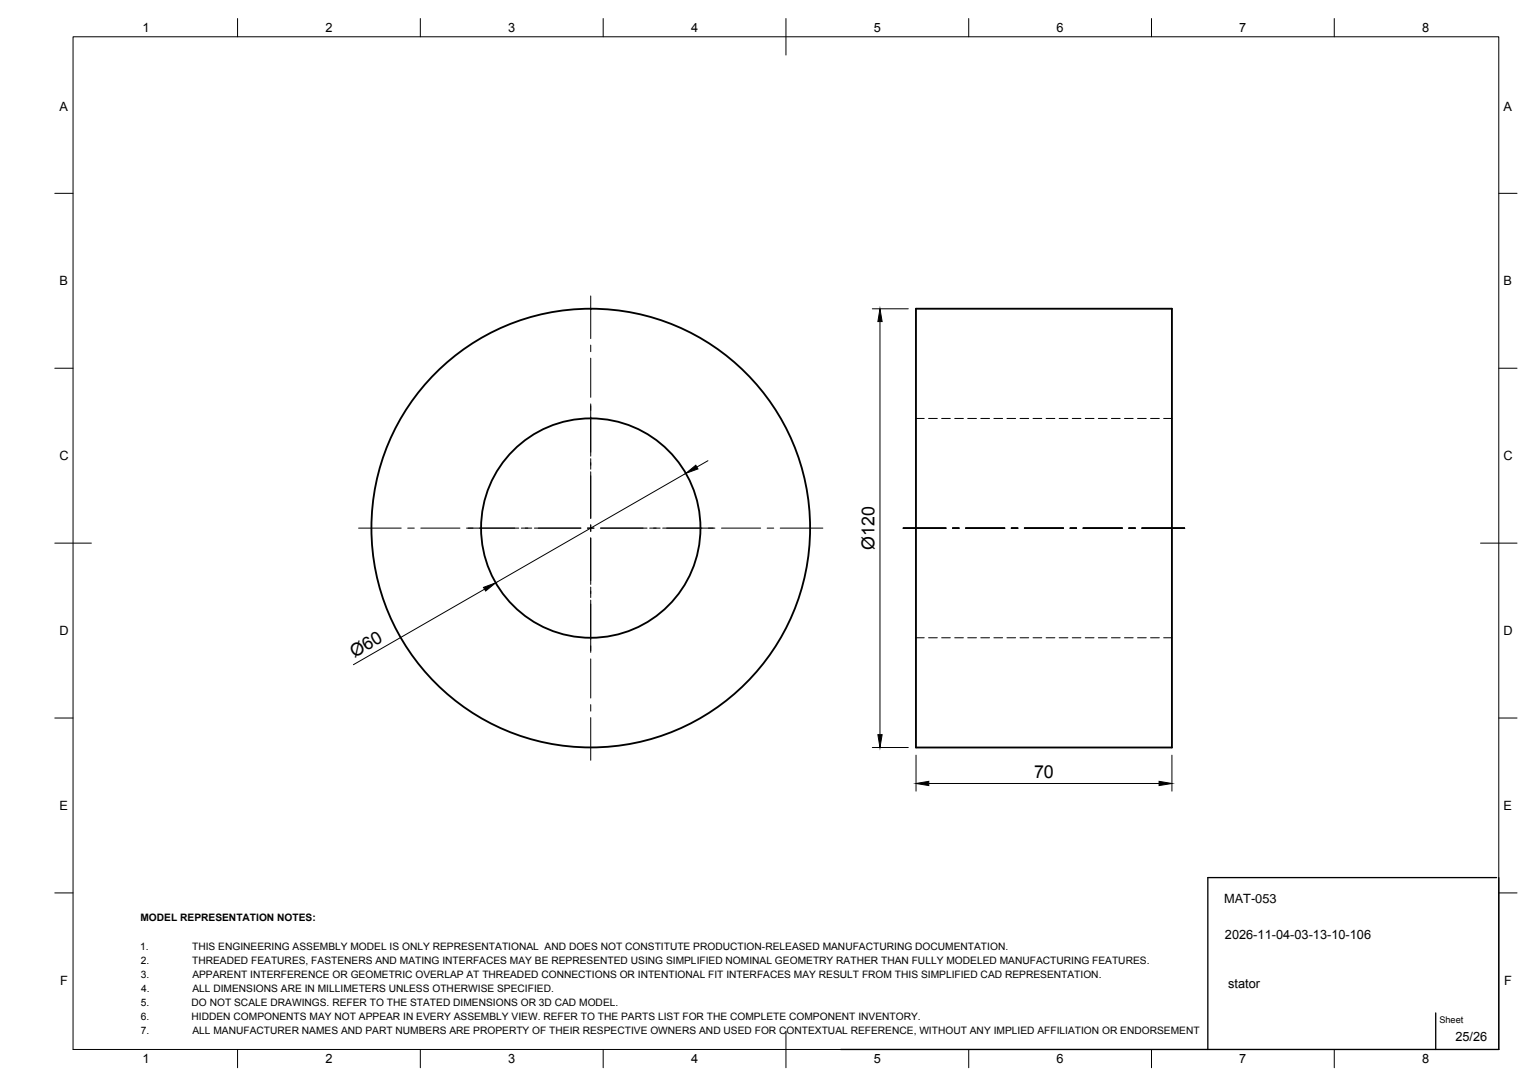
ISO-10303-21;
HEADER;
FILE_DESCRIPTION (('STEP AP214'),
    '1' );
FILE_NAME ('stator.step',
    '2026-10-10T03:43:58',
    ( '' ),
    ( '' ),
    'SwSTEP 2.0',
    'SolidWorks 2026',
    '' );
FILE_SCHEMA (( 'AUTOMOTIVE_DESIGN' ));
ENDSEC;

DATA;
#128=EDGE_CURVE ( 'NONE', #3129, #8050, #2808, .T. ) ;
#514=DIRECTION ( 'NONE',  ( 0.000000000000000000, 0.000000000000000000, -1.000000000000000000 ) ) ;
#771=EDGE_LOOP ( 'NONE', ( #32204, #20972 ) ) ;
#1378=ORIENTED_EDGE ( 'NONE', *, *, #27790, .F. ) ;
#2079=CARTESIAN_POINT ( 'NONE',  ( 0.000000000000000000, 70.00000000000000000, 0.000000000000000000 ) ) ;
#2691=DIRECTION ( 'NONE',  ( 0.000000000000000000, -0.000000000000000000, 1.000000000000000000 ) ) ;
#2808=LINE ( 'NONE', #13704, #47364 ) ;
#2968=ORIENTED_EDGE ( 'NONE', *, *, #54046, .T. ) ;
#3097=DIRECTION ( 'NONE',  ( 1.000000000000000000, 0.000000000000000000, 0.000000000000000000 ) ) ;
#3129=VERTEX_POINT ( 'NONE', #8923 ) ;
#3877=CARTESIAN_POINT ( 'NONE',  ( 0.000000000000000000, 70.00000000000000000, 0.000000000000000000 ) ) ;
#3906=VERTEX_POINT ( 'NONE', #13515 ) ;
#5010=PRODUCT_DEFINITION_CONTEXT ( 'detailed design', #48477, 'design' ) ;
#5620=SURFACE_STYLE_FILL_AREA ( #37284 ) ;
#6322=( NAMED_UNIT ( * ) SI_UNIT ( $, .STERADIAN. ) SOLID_ANGLE_UNIT ( ) );
#6922=DIRECTION ( 'NONE',  ( 0.000000000000000000, 0.000000000000000000, 1.000000000000000000 ) ) ;
#7111=DIRECTION ( 'NONE',  ( 0.000000000000000000, 1.000000000000000000, 0.000000000000000000 ) ) ;
#7237=ORIENTED_EDGE ( 'NONE', *, *, #40186, .F. ) ;
#7402=EDGE_CURVE ( 'NONE', #11928, #12092, #39946, .T. ) ;
#7531=CARTESIAN_POINT ( 'NONE',  ( 0.000000000000000000, 0.000000000000000000, -60.00000000000000000 ) ) ;
#8050=VERTEX_POINT ( 'NONE', #9236 ) ;
#8164=AXIS2_PLACEMENT_3D ( 'NONE', #38494, #11061, #514 ) ;
#8303=ORIENTED_EDGE ( 'NONE', *, *, #10070, .T. ) ;
#8319=DIRECTION ( 'NONE',  ( 1.000000000000000000, 0.000000000000000000, 0.000000000000000000 ) ) ;
#8479=CARTESIAN_POINT ( 'NONE',  ( 3.673940397442059178E-15, 70.00000000000000000, 30.00000000000000000 ) ) ;
#8923=CARTESIAN_POINT ( 'NONE',  ( 7.347880794884118356E-15, 70.00000000000000000, 60.00000000000000000 ) ) ;
#9236=CARTESIAN_POINT ( 'NONE',  ( 7.347880794884118356E-15, 0.000000000000000000, 60.00000000000000000 ) ) ;
#10070=EDGE_CURVE ( 'NONE', #11364, #8050, #65973, .T. ) ;
#10554=FILL_AREA_STYLE_COLOUR ( '', #23478 ) ;
#10805=PRODUCT_DEFINITION_FORMATION_WITH_SPECIFIED_SOURCE ( 'ANY', '', #45703, .NOT_KNOWN. ) ;
#11061=DIRECTION ( 'NONE',  ( -0.000000000000000000, -1.000000000000000000, -0.000000000000000000 ) ) ;
#11364=VERTEX_POINT ( 'NONE', #7531 ) ;
#11398=CYLINDRICAL_SURFACE ( 'NONE', #8164, 60.00000000000000000 ) ;
#11411=CLOSED_SHELL ( 'NONE', ( #11814, #48594, #51527, #41201, #53636, #22060 ) ) ;
#11814=ADVANCED_FACE ( 'NONE', ( #47465 ), #57354, .F. ) ;
#11928=VERTEX_POINT ( 'NONE', #8479 ) ;
#12092=VERTEX_POINT ( 'NONE', #18597 ) ;
#12606=ORIENTED_EDGE ( 'NONE', *, *, #34401, .T. ) ;
#13254=FACE_OUTER_BOUND ( 'NONE', #69197, .T. ) ;
#13515=CARTESIAN_POINT ( 'NONE',  ( 0.000000000000000000, 70.00000000000000000, -60.00000000000000000 ) ) ;
#13591=DIRECTION ( 'NONE',  ( 0.000000000000000000, 1.000000000000000000, 0.000000000000000000 ) ) ;
#13704=CARTESIAN_POINT ( 'NONE',  ( 7.347880794884118356E-15, 70.00000000000000000, 60.00000000000000000 ) ) ;
#13722=DIRECTION ( 'NONE',  ( 0.000000000000000000, 1.000000000000000000, 0.000000000000000000 ) ) ;
#14303=ORIENTED_EDGE ( 'NONE', *, *, #34401, .F. ) ;
#14387=CARTESIAN_POINT ( 'NONE',  ( 0.000000000000000000, 70.00000000000000000, -30.00000000000000000 ) ) ;
#15284=DIRECTION ( 'NONE',  ( 0.000000000000000000, 1.000000000000000000, 0.000000000000000000 ) ) ;
#15336=EDGE_CURVE ( 'NONE', #12092, #11928, #55552, .T. ) ;
#16532=AXIS2_PLACEMENT_3D ( 'NONE', #62277, #31318, #62972 ) ;
#16657=AXIS2_PLACEMENT_3D ( 'NONE', #26661, #63948, #26322 ) ;
#17905=AXIS2_PLACEMENT_3D ( 'NONE', #34759, #57593, #3097 ) ;
#17988=ORIENTED_EDGE ( 'NONE', *, *, #58843, .T. ) ;
#18093=( LENGTH_UNIT ( ) NAMED_UNIT ( * ) SI_UNIT ( .MILLI., .METRE. ) );
#18597=CARTESIAN_POINT ( 'NONE',  ( 0.000000000000000000, 70.00000000000000000, -30.00000000000000000 ) ) ;
#19703=( GEOMETRIC_REPRESENTATION_CONTEXT ( 3 ) GLOBAL_UNCERTAINTY_ASSIGNED_CONTEXT ( ( #55717 ) ) GLOBAL_UNIT_ASSIGNED_CONTEXT ( ( #18093, #66306, #23020 ) ) REPRESENTATION_CONTEXT ( 'NONE', 'WORKASPACE' ) );
#19882=EDGE_LOOP ( 'NONE', ( #42252, #31669, #65286, #8303 ) ) ;
#19919=EDGE_LOOP ( 'NONE', ( #40783, #67233 ) ) ;
#20062=ORIENTED_EDGE ( 'NONE', *, *, #128, .T. ) ;
#20100=MECHANICAL_DESIGN_GEOMETRIC_PRESENTATION_REPRESENTATION('',(#40332),#38058);
#20972=ORIENTED_EDGE ( 'NONE', *, *, #7402, .F. ) ;
#21799=PRESENTATION_STYLE_ASSIGNMENT (( #53454 ) ) ;
#22060=ADVANCED_FACE ( 'NONE', ( #55522 ), #50256, .F. ) ;
#23020=( NAMED_UNIT ( * ) SI_UNIT ( $, .STERADIAN. ) SOLID_ANGLE_UNIT ( ) );
#23025=AXIS2_PLACEMENT_3D ( 'NONE', #33668, #55448, #6922 ) ;
#23478=COLOUR_RGB ( '',0.7921568627450980005, 0.8196078431372548767, 0.9333333333333333481 ) ;
#23530=DIRECTION ( 'NONE',  ( -0.000000000000000000, -1.000000000000000000, -0.000000000000000000 ) ) ;
#23730=DIRECTION ( 'NONE',  ( -0.000000000000000000, -1.000000000000000000, -0.000000000000000000 ) ) ;
#25005=LINE ( 'NONE', #35552, #56810 ) ;
#25560=VERTEX_POINT ( 'NONE', #41893 ) ;
#25651=ORIENTED_EDGE ( 'NONE', *, *, #27790, .T. ) ;
#26071=CARTESIAN_POINT ( 'NONE',  ( 3.673940397442059178E-15, 0.000000000000000000, 30.00000000000000000 ) ) ;
#26322=DIRECTION ( 'NONE',  ( 0.000000000000000000, 0.000000000000000000, -1.000000000000000000 ) ) ;
#26661=CARTESIAN_POINT ( 'NONE',  ( 0.000000000000000000, 70.00000000000000000, 0.000000000000000000 ) ) ;
#26809=ORIENTED_EDGE ( 'NONE', *, *, #49285, .F. ) ;
#27752=AXIS2_PLACEMENT_3D ( 'NONE', #29958, #7111, #51420 ) ;
#27790=EDGE_CURVE ( 'NONE', #11928, #65701, #25005, .T. ) ;
#28733=PLANE ( 'NONE',  #66663 ) ;
#29336=SHAPE_REPRESENTATION_RELATIONSHIP ( 'NONE' , 'NONE' ,  #38847, #62542 ) ;
#29349=LINE ( 'NONE', #61013, #40185 ) ;
#29675=UNCERTAINTY_MEASURE_WITH_UNIT (LENGTH_MEASURE( 1.000000000000000082E-05 ), #49218, 'distance_accuracy_value', 'NONE');
#29958=CARTESIAN_POINT ( 'NONE',  ( 0.000000000000000000, 0.000000000000000000, 0.000000000000000000 ) ) ;
#30601=CARTESIAN_POINT ( 'NONE',  ( 0.000000000000000000, 70.00000000000000000, 0.000000000000000000 ) ) ;
#31318=DIRECTION ( 'NONE',  ( -0.000000000000000000, -1.000000000000000000, -0.000000000000000000 ) ) ;
#31350=EDGE_CURVE ( 'NONE', #3906, #11364, #29349, .T. ) ;
#31410=CIRCLE ( 'NONE', #17905, 60.00000000000000000 ) ;
#31669=ORIENTED_EDGE ( 'NONE', *, *, #52351, .F. ) ;
#31674=( NAMED_UNIT ( * ) PLANE_ANGLE_UNIT ( ) SI_UNIT ( $, .RADIAN. ) );
#32204=ORIENTED_EDGE ( 'NONE', *, *, #15336, .F. ) ;
#32372=SURFACE_SIDE_STYLE ('',( #5620 ) ) ;
#32497=CARTESIAN_POINT ( 'NONE',  ( 0.000000000000000000, 0.000000000000000000, 0.000000000000000000 ) ) ;
#32994=CIRCLE ( 'NONE', #47593, 30.00000000000000000 ) ;
#33668=CARTESIAN_POINT ( 'NONE',  ( 0.000000000000000000, 70.00000000000000000, 0.000000000000000000 ) ) ;
#34275=CIRCLE ( 'NONE', #66872, 60.00000000000000000 ) ;
#34401=EDGE_CURVE ( 'NONE', #3129, #3906, #31410, .T. ) ;
#34759=CARTESIAN_POINT ( 'NONE',  ( 0.000000000000000000, 70.00000000000000000, 0.000000000000000000 ) ) ;
#35552=CARTESIAN_POINT ( 'NONE',  ( 3.673940397442059178E-15, 70.00000000000000000, 30.00000000000000000 ) ) ;
#36639=ORIENTED_EDGE ( 'NONE', *, *, #31350, .F. ) ;
#36743=CARTESIAN_POINT ( 'NONE',  ( 0.000000000000000000, 0.000000000000000000, 0.000000000000000000 ) ) ;
#36757=CIRCLE ( 'NONE', #27752, 30.00000000000000000 ) ;
#36786=AXIS2_PLACEMENT_3D ( 'NONE', #36743, #15284, #62438 ) ;
#36923=DIRECTION ( 'NONE',  ( 1.000000000000000000, 0.000000000000000000, 0.000000000000000000 ) ) ;
#37284=FILL_AREA_STYLE ('',( #10554 ) ) ;
#37524=CARTESIAN_POINT ( 'NONE',  ( 0.000000000000000000, 0.000000000000000000, 0.000000000000000000 ) ) ;
#37638=ORIENTED_EDGE ( 'NONE', *, *, #15336, .T. ) ;
#38058=( GEOMETRIC_REPRESENTATION_CONTEXT ( 3 ) GLOBAL_UNCERTAINTY_ASSIGNED_CONTEXT ( ( #29675 ) ) GLOBAL_UNIT_ASSIGNED_CONTEXT ( ( #49218, #31674, #6322 ) ) REPRESENTATION_CONTEXT ( 'NONE', 'WORKASPACE' ) );
#38494=CARTESIAN_POINT ( 'NONE',  ( 0.000000000000000000, 70.00000000000000000, 0.000000000000000000 ) ) ;
#38847=SHAPE_REPRESENTATION ( 'stator', ( #66832 ), #19703 ) ;
#38996=ORIENTED_EDGE ( 'NONE', *, *, #7402, .T. ) ;
#39079=FACE_OUTER_BOUND ( 'NONE', #44402, .T. ) ;
#39696=VECTOR ( 'NONE', #50973, 1000.000000000000000 ) ;
#39764=PLANE ( 'NONE',  #42835 ) ;
#39946=CIRCLE ( 'NONE', #59011, 30.00000000000000000 ) ;
#40136=DIRECTION ( 'NONE',  ( -0.000000000000000000, -1.000000000000000000, -0.000000000000000000 ) ) ;
#40185=VECTOR ( 'NONE', #23730, 1000.000000000000000 ) ;
#40186=EDGE_CURVE ( 'NONE', #65701, #25560, #32994, .T. ) ;
#40332=STYLED_ITEM ( 'NONE', ( #21799 ), #64301 ) ;
#40783=ORIENTED_EDGE ( 'NONE', *, *, #49285, .T. ) ;
#41023=SHAPE_DEFINITION_REPRESENTATION ( #55202, #38847 ) ;
#41201=ADVANCED_FACE ( 'NONE', ( #13254, #61086 ), #28733, .F. ) ;
#41893=CARTESIAN_POINT ( 'NONE',  ( 0.000000000000000000, 0.000000000000000000, -30.00000000000000000 ) ) ;
#42252=ORIENTED_EDGE ( 'NONE', *, *, #128, .F. ) ;
#42699=DIRECTION ( 'NONE',  ( 0.000000000000000000, 1.000000000000000000, 0.000000000000000000 ) ) ;
#42835=AXIS2_PLACEMENT_3D ( 'NONE', #65818, #13722, #50660 ) ;
#43080=PRODUCT_DEFINITION ( 'UNKNOWN', '', #10805, #5010 ) ;
#43081=AXIS2_PLACEMENT_3D ( 'NONE', #2079, #23530, #45318 ) ;
#43167=CYLINDRICAL_SURFACE ( 'NONE', #16657, 60.00000000000000000 ) ;
#43193=ORIENTED_EDGE ( 'NONE', *, *, #54046, .F. ) ;
#44402=EDGE_LOOP ( 'NONE', ( #67755, #12606 ) ) ;
#44558=DIRECTION ( 'NONE',  ( 0.000000000000000000, 0.000000000000000000, 1.000000000000000000 ) ) ;
#44655=ORIENTED_EDGE ( 'NONE', *, *, #10070, .F. ) ;
#45318=DIRECTION ( 'NONE',  ( 0.000000000000000000, 0.000000000000000000, -1.000000000000000000 ) ) ;
#45703=PRODUCT ( 'stator', 'stator', '', ( #47664 ) ) ;
#46417=EDGE_LOOP ( 'NONE', ( #37638, #25651, #26809, #43193 ) ) ;
#47364=VECTOR ( 'NONE', #67195, 1000.000000000000000 ) ;
#47465=FACE_OUTER_BOUND ( 'NONE', #46417, .T. ) ;
#47593=AXIS2_PLACEMENT_3D ( 'NONE', #37524, #65310, #54384 ) ;
#47664=PRODUCT_CONTEXT ( 'NONE', #66008, 'mechanical' ) ;
#47809=DIRECTION ( 'NONE',  ( 0.000000000000000000, 1.000000000000000000, 0.000000000000000000 ) ) ;
#48477=APPLICATION_CONTEXT ( 'automotive_design' ) ;
#48496=CIRCLE ( 'NONE', #57529, 60.00000000000000000 ) ;
#48594=ADVANCED_FACE ( 'NONE', ( #53723 ), #43167, .T. ) ;
#49218=( LENGTH_UNIT ( ) NAMED_UNIT ( * ) SI_UNIT ( .MILLI., .METRE. ) );
#49285=EDGE_CURVE ( 'NONE', #25560, #65701, #36757, .T. ) ;
#50256=CYLINDRICAL_SURFACE ( 'NONE', #43081, 30.00000000000000000 ) ;
#50530=CARTESIAN_POINT ( 'NONE',  ( 0.000000000000000000, 0.000000000000000000, 0.000000000000000000 ) ) ;
#50660=DIRECTION ( 'NONE',  ( 0.000000000000000000, -0.000000000000000000, 1.000000000000000000 ) ) ;
#50973=DIRECTION ( 'NONE',  ( -0.000000000000000000, -1.000000000000000000, -0.000000000000000000 ) ) ;
#51420=DIRECTION ( 'NONE',  ( 0.000000000000000000, 0.000000000000000000, 1.000000000000000000 ) ) ;
#51527=ADVANCED_FACE ( 'NONE', ( #39079, #55588 ), #39764, .T. ) ;
#52351=EDGE_CURVE ( 'NONE', #3906, #3129, #48496, .T. ) ;
#53454=SURFACE_STYLE_USAGE ( .BOTH. , #32372 ) ;
#53588=DIRECTION ( 'NONE',  ( 1.000000000000000000, 0.000000000000000000, 0.000000000000000000 ) ) ;
#53636=ADVANCED_FACE ( 'NONE', ( #65953 ), #11398, .T. ) ;
#53723=FACE_OUTER_BOUND ( 'NONE', #67488, .T. ) ;
#54046=EDGE_CURVE ( 'NONE', #12092, #25560, #56950, .T. ) ;
#54384=DIRECTION ( 'NONE',  ( 0.000000000000000000, 0.000000000000000000, 1.000000000000000000 ) ) ;
#55202=PRODUCT_DEFINITION_SHAPE ( 'NONE', 'NONE',  #43080 ) ;
#55448=DIRECTION ( 'NONE',  ( 0.000000000000000000, 1.000000000000000000, 0.000000000000000000 ) ) ;
#55522=FACE_OUTER_BOUND ( 'NONE', #66699, .T. ) ;
#55552=CIRCLE ( 'NONE', #23025, 30.00000000000000000 ) ;
#55588=FACE_BOUND ( 'NONE', #771, .T. ) ;
#55717=UNCERTAINTY_MEASURE_WITH_UNIT (LENGTH_MEASURE( 1.000000000000000082E-05 ), #18093, 'distance_accuracy_value', 'NONE');
#56635=DIRECTION ( 'NONE',  ( 0.000000000000000000, 1.000000000000000000, 0.000000000000000000 ) ) ;
#56810=VECTOR ( 'NONE', #40136, 1000.000000000000000 ) ;
#56950=LINE ( 'NONE', #14387, #39696 ) ;
#57354=CYLINDRICAL_SURFACE ( 'NONE', #16532, 30.00000000000000000 ) ;
#57529=AXIS2_PLACEMENT_3D ( 'NONE', #3877, #47809, #36923 ) ;
#57593=DIRECTION ( 'NONE',  ( 0.000000000000000000, 1.000000000000000000, 0.000000000000000000 ) ) ;
#58843=EDGE_CURVE ( 'NONE', #8050, #11364, #34275, .T. ) ;
#59011=AXIS2_PLACEMENT_3D ( 'NONE', #30601, #56635, #66866 ) ;
#59446=ORIENTED_EDGE ( 'NONE', *, *, #58843, .F. ) ;
#61013=CARTESIAN_POINT ( 'NONE',  ( 0.000000000000000000, 70.00000000000000000, -60.00000000000000000 ) ) ;
#61086=FACE_BOUND ( 'NONE', #19919, .T. ) ;
#61765=CARTESIAN_POINT ( 'NONE',  ( 0.000000000000000000, 0.000000000000000000, 0.000000000000000000 ) ) ;
#62277=CARTESIAN_POINT ( 'NONE',  ( 0.000000000000000000, 70.00000000000000000, 0.000000000000000000 ) ) ;
#62438=DIRECTION ( 'NONE',  ( 1.000000000000000000, 0.000000000000000000, 0.000000000000000000 ) ) ;
#62542=ADVANCED_BREP_SHAPE_REPRESENTATION ( '', ( #64301, #66832 ), #19703 ) ;
#62972=DIRECTION ( 'NONE',  ( 0.000000000000000000, 0.000000000000000000, -1.000000000000000000 ) ) ;
#63948=DIRECTION ( 'NONE',  ( -0.000000000000000000, -1.000000000000000000, -0.000000000000000000 ) ) ;
#64301=MANIFOLD_SOLID_BREP ( 'Extrude-Thin1', #11411 ) ;
#65286=ORIENTED_EDGE ( 'NONE', *, *, #31350, .T. ) ;
#65310=DIRECTION ( 'NONE',  ( 0.000000000000000000, 1.000000000000000000, 0.000000000000000000 ) ) ;
#65701=VERTEX_POINT ( 'NONE', #26071 ) ;
#65818=CARTESIAN_POINT ( 'NONE',  ( 0.000000000000000000, 70.00000000000000000, 0.000000000000000000 ) ) ;
#65953=FACE_OUTER_BOUND ( 'NONE', #19882, .T. ) ;
#65973=CIRCLE ( 'NONE', #36786, 60.00000000000000000 ) ;
#66008=APPLICATION_CONTEXT ( 'automotive_design' ) ;
#66306=( NAMED_UNIT ( * ) PLANE_ANGLE_UNIT ( ) SI_UNIT ( $, .RADIAN. ) );
#66663=AXIS2_PLACEMENT_3D ( 'NONE', #61765, #13591, #2691 ) ;
#66699=EDGE_LOOP ( 'NONE', ( #1378, #38996, #2968, #7237 ) ) ;
#66832=AXIS2_PLACEMENT_3D ( 'NONE', #50530, #44558, #8319 ) ;
#66866=DIRECTION ( 'NONE',  ( 0.000000000000000000, 0.000000000000000000, 1.000000000000000000 ) ) ;
#66872=AXIS2_PLACEMENT_3D ( 'NONE', #32497, #42699, #53588 ) ;
#67195=DIRECTION ( 'NONE',  ( -0.000000000000000000, -1.000000000000000000, -0.000000000000000000 ) ) ;
#67233=ORIENTED_EDGE ( 'NONE', *, *, #40186, .T. ) ;
#67488=EDGE_LOOP ( 'NONE', ( #14303, #20062, #17988, #36639 ) ) ;
#67755=ORIENTED_EDGE ( 'NONE', *, *, #52351, .T. ) ;
#69197=EDGE_LOOP ( 'NONE', ( #44655, #59446 ) ) ;
ENDSEC;
END-ISO-10303-21;
